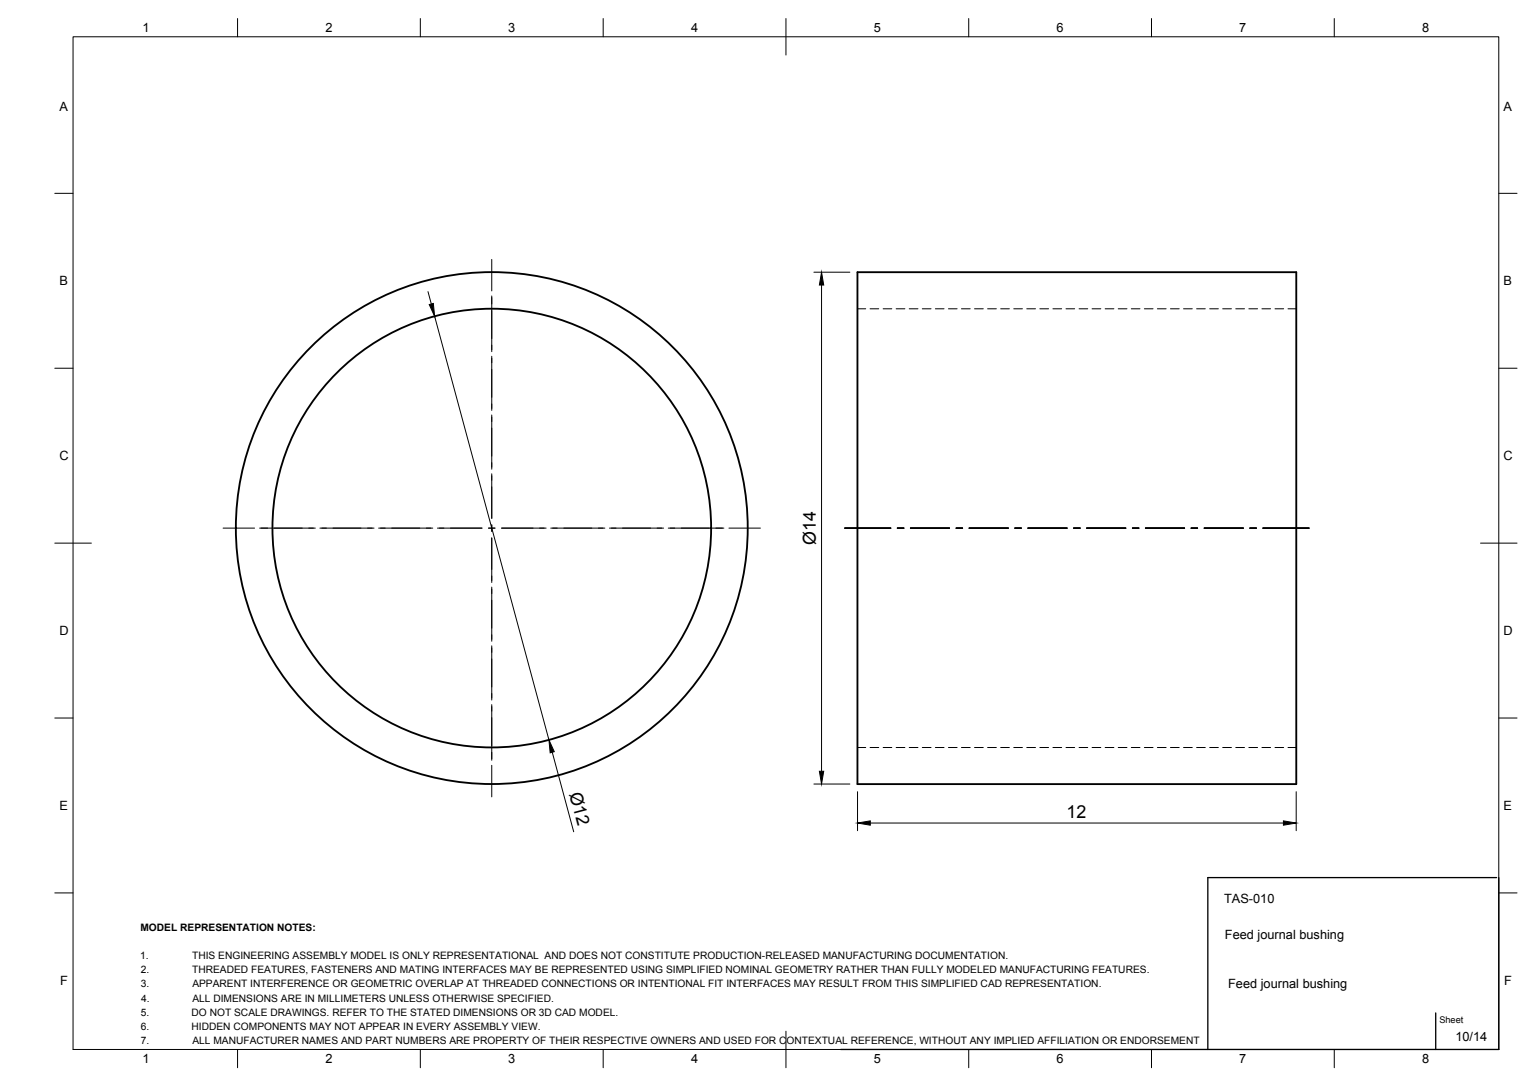
ISO-10303-21;
HEADER;
/* Generated by software containing ST-Developer
 * from STEP Tools, Inc. (www.steptools.com) 
 */

FILE_DESCRIPTION(
/* description */ (
'Independent keyed-quill tailstock, native coupled50mm slider andM16x2
 feed screw, conical dead center, bronze sleeves/thrust washers, cross
-pinned handwheel and bolted guide key. Custom center taper; no standa
rd taper compatibility, machine-bed compatibility or load rating assig
ned.'),
/* implementation_level */ '2;1');

FILE_NAME(
/* name */ 'Feed journal bushing.step',
/* time_stamp */ '2026-11-14T07:17:36-08:00',
/* author */ (''),
/* organization */ (''),
/* preprocessor_version */ 'ST-DEVELOPER v20.2',
/* originating_system */ 'Autodesk Translation Framework v15.17.0.0',
/* authorisation */ '');

FILE_SCHEMA (('AUTOMOTIVE_DESIGN { 1 0 10303 214 3 1 1 }'));
ENDSEC;

DATA;
#10=MECHANICAL_DESIGN_GEOMETRIC_PRESENTATION_REPRESENTATION('',(#160),#289387);
#126=SHAPE_REPRESENTATION_RELATIONSHIP('SRR','None',#289461,#143);
#143=ADVANCED_BREP_SHAPE_REPRESENTATION('',(#177),#289377);
#160=STYLED_ITEM('',(#289550),#177);
#177=MANIFOLD_SOLID_BREP('Body1',#16848);
#238=FACE_BOUND('',#1566,.T.);
#239=FACE_BOUND('',#1568,.T.);
#371=PLANE('',#17582);
#372=PLANE('',#17583);
#862=FACE_OUTER_BOUND('',#1563,.T.);
#863=FACE_OUTER_BOUND('',#1564,.T.);
#864=FACE_OUTER_BOUND('',#1565,.T.);
#865=FACE_OUTER_BOUND('',#1567,.T.);
#1563=EDGE_LOOP('',(#13787,#13788,#13789,#13790));
#1564=EDGE_LOOP('',(#13791,#13792,#13793,#13794));
#1565=EDGE_LOOP('',(#13795));
#1566=EDGE_LOOP('',(#13796));
#1567=EDGE_LOOP('',(#13797));
#1568=EDGE_LOOP('',(#13798));
#1913=CIRCLE('',#17577,6.);
#1914=CIRCLE('',#17578,6.);
#1915=CIRCLE('',#17580,7.);
#1916=CIRCLE('',#17581,7.);
#4372=LINE('',#185290,#5009);
#4373=LINE('',#185296,#5010);
#5009=VECTOR('',#19384,6.);
#5010=VECTOR('',#19391,7.);
#6618=VERTEX_POINT('',#185287);
#6619=VERTEX_POINT('',#185289);
#6620=VERTEX_POINT('',#185293);
#6621=VERTEX_POINT('',#185295);
#9205=EDGE_CURVE('',#6618,#6618,#1913,.T.);
#9206=EDGE_CURVE('',#6618,#6619,#4372,.T.);
#9207=EDGE_CURVE('',#6619,#6619,#1914,.T.);
#9208=EDGE_CURVE('',#6620,#6620,#1915,.T.);
#9209=EDGE_CURVE('',#6620,#6621,#4373,.T.);
#9210=EDGE_CURVE('',#6621,#6621,#1916,.T.);
#13787=ORIENTED_EDGE('',*,*,#9205,.T.);
#13788=ORIENTED_EDGE('',*,*,#9206,.T.);
#13789=ORIENTED_EDGE('',*,*,#9207,.F.);
#13790=ORIENTED_EDGE('',*,*,#9206,.F.);
#13791=ORIENTED_EDGE('',*,*,#9208,.F.);
#13792=ORIENTED_EDGE('',*,*,#9209,.T.);
#13793=ORIENTED_EDGE('',*,*,#9210,.T.);
#13794=ORIENTED_EDGE('',*,*,#9209,.F.);
#13795=ORIENTED_EDGE('',*,*,#9208,.T.);
#13796=ORIENTED_EDGE('',*,*,#9207,.T.);
#13797=ORIENTED_EDGE('',*,*,#9210,.F.);
#13798=ORIENTED_EDGE('',*,*,#9205,.F.);
#16045=CYLINDRICAL_SURFACE('',#17576,6.);
#16046=CYLINDRICAL_SURFACE('',#17579,7.);
#16630=ADVANCED_FACE('',(#862),#16045,.F.);
#16631=ADVANCED_FACE('',(#863),#16046,.T.);
#16632=ADVANCED_FACE('',(#864,#238),#371,.T.);
#16633=ADVANCED_FACE('',(#865,#239),#372,.F.);
#16848=CLOSED_SHELL('',(#16630,#16631,#16632,#16633));
#17575=AXIS2_PLACEMENT_3D('',#185285,#19378,#19379);
#17576=AXIS2_PLACEMENT_3D('',#185286,#19380,#19381);
#17577=AXIS2_PLACEMENT_3D('',#185288,#19382,#19383);
#17578=AXIS2_PLACEMENT_3D('',#185291,#19385,#19386);
#17579=AXIS2_PLACEMENT_3D('',#185292,#19387,#19388);
#17580=AXIS2_PLACEMENT_3D('',#185294,#19389,#19390);
#17581=AXIS2_PLACEMENT_3D('',#185297,#19392,#19393);
#17582=AXIS2_PLACEMENT_3D('',#185298,#19394,#19395);
#17583=AXIS2_PLACEMENT_3D('',#185299,#19396,#19397);
#19378=DIRECTION('axis',(0.,0.,1.));
#19379=DIRECTION('refdir',(1.,0.,0.));
#19380=DIRECTION('center_axis',(0.,0.,1.));
#19381=DIRECTION('ref_axis',(1.,0.,0.));
#19382=DIRECTION('center_axis',(0.,0.,-1.));
#19383=DIRECTION('ref_axis',(1.,0.,0.));
#19384=DIRECTION('',(0.,0.,1.));
#19385=DIRECTION('center_axis',(0.,0.,-1.));
#19386=DIRECTION('ref_axis',(1.,0.,0.));
#19387=DIRECTION('center_axis',(0.,0.,1.));
#19388=DIRECTION('ref_axis',(1.,0.,0.));
#19389=DIRECTION('center_axis',(0.,0.,1.));
#19390=DIRECTION('ref_axis',(1.,0.,0.));
#19391=DIRECTION('',(0.,0.,-1.));
#19392=DIRECTION('center_axis',(0.,0.,1.));
#19393=DIRECTION('ref_axis',(1.,0.,0.));
#19394=DIRECTION('center_axis',(0.,0.,1.));
#19395=DIRECTION('ref_axis',(1.,0.,0.));
#19396=DIRECTION('center_axis',(0.,0.,1.));
#19397=DIRECTION('ref_axis',(1.,0.,0.));
#185285=CARTESIAN_POINT('',(0.,0.,0.));
#185286=CARTESIAN_POINT('Origin',(0.,0.,0.));
#185287=CARTESIAN_POINT('',(-6.,-7.34788079488412E-16,0.));
#185288=CARTESIAN_POINT('Origin',(0.,0.,0.));
#185289=CARTESIAN_POINT('',(-6.,-7.34788079488412E-16,12.));
#185290=CARTESIAN_POINT('',(-6.,-7.34788079488412E-16,0.));
#185291=CARTESIAN_POINT('Origin',(0.,0.,12.));
#185292=CARTESIAN_POINT('Origin',(0.,0.,0.));
#185293=CARTESIAN_POINT('',(-7.,-8.57252759403147E-16,12.));
#185294=CARTESIAN_POINT('Origin',(0.,0.,12.));
#185295=CARTESIAN_POINT('',(-7.,-8.57252759403147E-16,0.));
#185296=CARTESIAN_POINT('',(-7.,-8.57252759403147E-16,0.));
#185297=CARTESIAN_POINT('Origin',(0.,0.,0.));
#185298=CARTESIAN_POINT('Origin',(0.,0.,12.));
#185299=CARTESIAN_POINT('Origin',(0.,0.,0.));
#289358=UNCERTAINTY_MEASURE_WITH_UNIT(LENGTH_MEASURE(0.01),#289388,
'DISTANCE_ACCURACY_VALUE',
'Maximum model space distance between geometric entities at asserted c
onnectivities');
#289368=UNCERTAINTY_MEASURE_WITH_UNIT(LENGTH_MEASURE(0.01),#289388,
'DISTANCE_ACCURACY_VALUE',
'Maximum model space distance between geometric entities at asserted c
onnectivities');
#289377=(
GEOMETRIC_REPRESENTATION_CONTEXT(3)
GLOBAL_UNCERTAINTY_ASSIGNED_CONTEXT((#289358))
GLOBAL_UNIT_ASSIGNED_CONTEXT((#289388,#289390,#289391))
REPRESENTATION_CONTEXT('','3D')
);
#289387=(
GEOMETRIC_REPRESENTATION_CONTEXT(3)
GLOBAL_UNCERTAINTY_ASSIGNED_CONTEXT((#289368))
GLOBAL_UNIT_ASSIGNED_CONTEXT((#289388,#289390,#289391))
REPRESENTATION_CONTEXT('','3D')
);
#289388=(
LENGTH_UNIT()
NAMED_UNIT(*)
SI_UNIT(.MILLI.,.METRE.)
);
#289390=(
NAMED_UNIT(*)
PLANE_ANGLE_UNIT()
SI_UNIT($,.RADIAN.)
);
#289391=(
NAMED_UNIT(*)
SI_UNIT($,.STERADIAN.)
SOLID_ANGLE_UNIT()
);
#289400=SHAPE_DEFINITION_REPRESENTATION(#289418,#289461);
#289418=PRODUCT_DEFINITION_SHAPE('',$,#289480);
#289461=SHAPE_REPRESENTATION('',(#17575),#289377);
#289471=PRODUCT_DEFINITION_CONTEXT('part definition',#289527,'design');
#289480=PRODUCT_DEFINITION('Feed journal bushing',
'Feed journal bushing',#289498,#289471);
#289498=PRODUCT_DEFINITION_FORMATION('',$,#289537);
#289527=APPLICATION_CONTEXT(
'Core Data for Automotive Mechanical Design Process');
#289528=PRODUCT_CONTEXT('part definition',#289527,'mechanical');
#289537=PRODUCT('Feed journal bushing','Feed journal bushing',$,(#289528));
#289550=PRESENTATION_STYLE_ASSIGNMENT((#289557));
#289557=SURFACE_STYLE_USAGE(.BOTH.,#289564);
#289564=SURFACE_SIDE_STYLE('',(#289571));
#289571=SURFACE_STYLE_FILL_AREA(#289578);
#289578=FILL_AREA_STYLE('Opaque(185,192,202)',(#289585));
#289585=FILL_AREA_STYLE_COLOUR('Opaque(185,192,202)',#289592);
#289592=COLOUR_RGB('Opaque(185,192,202)',0.725490196078431,0.752941176470588,
0.792156862745098);
ENDSEC;
END-ISO-10303-21;
